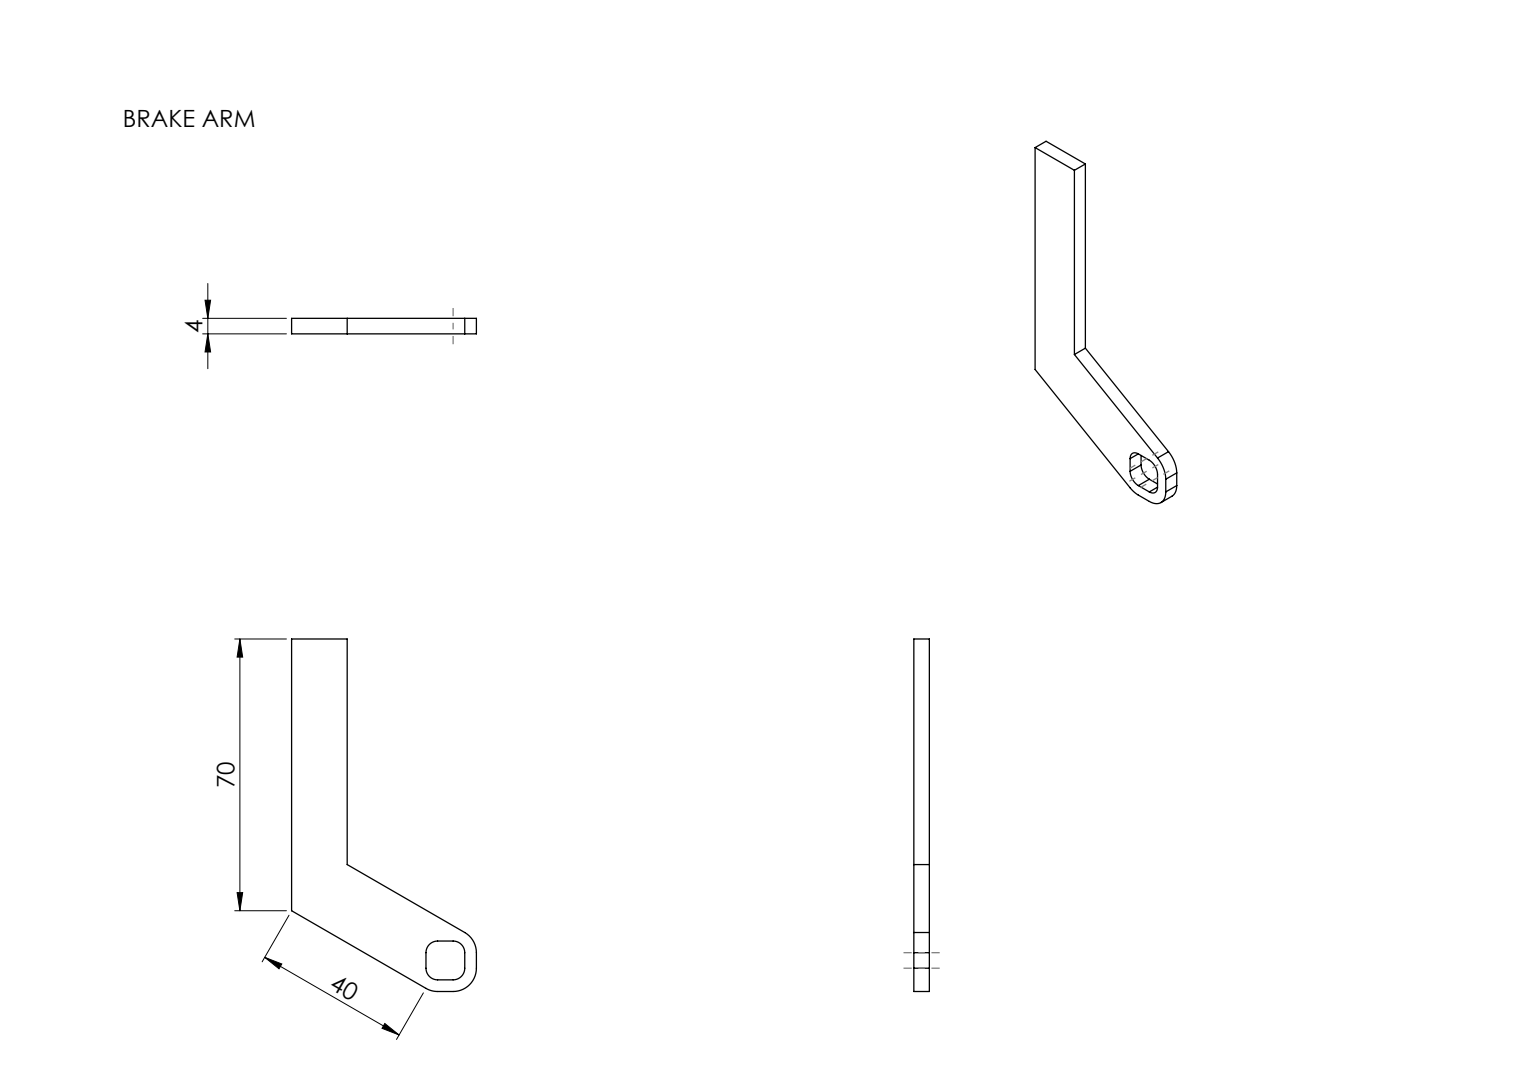
ISO-10303-21;
HEADER;
FILE_DESCRIPTION (('STEP AP214'),
    '1' );
FILE_NAME ('brake arm.step',
    '2026-10-08T05:56:58',
    ( '' ),
    ( '' ),
    'SwSTEP 2.0',
    'SolidWorks 2026',
    '' );
FILE_SCHEMA (( 'AUTOMOTIVE_DESIGN' ));
ENDSEC;

DATA;
#81=AXIS2_PLACEMENT_3D ( 'NONE', #18484, #1485, #6266 ) ;
#85=ORIENTED_EDGE ( 'NONE', *, *, #1576, .T. ) ;
#161=EDGE_LOOP ( 'NONE', ( #14576, #14310, #4192, #11228 ) ) ;
#198=CARTESIAN_POINT ( 'NONE',  ( -2.000000000000000000, 1.999999999999998224, 41.99999999999999289 ) ) ;
#237=EDGE_CURVE ( 'NONE', #6503, #6248, #1744, .T. ) ;
#247=VECTOR ( 'NONE', #10712, 1000.000000000000000 ) ;
#276=EDGE_CURVE ( 'NONE', #11279, #870, #9053, .T. ) ;
#316=CARTESIAN_POINT ( 'NONE',  ( -25.31088913245550032, 24.69615242270646149, 37.99999999999999289 ) ) ;
#333=EDGE_CURVE ( 'NONE', #18696, #7394, #11045, .T. ) ;
#336=COLOUR_RGB ( '', 0.08235294, 0.09019608, 0.10196078) ;
#393=VECTOR ( 'NONE', #16004, 1000.000000000000000 ) ;
#399=EDGE_CURVE ( 'NONE', #17067, #16866, #445, .T. ) ;
#445=LINE ( 'NONE', #1934, #5840 ) ;
#469=AXIS2_PLACEMENT_3D ( 'NONE', #3938, #11542, #11357 ) ;
#506=ORIENTED_EDGE ( 'NONE', *, *, #18779, .F. ) ;
#580=CARTESIAN_POINT ( 'NONE',  ( 5.000000000000000000, 1.999999999999998224, 37.99999999999999289 ) ) ;
#596=CIRCLE ( 'NONE', #10178, 3.000000000000000000 ) ;
#602=CARTESIAN_POINT ( 'NONE',  ( -39.64101615137757761, -1.650388831904890594E-13, 37.99999999999999289 ) ) ;
#648=CARTESIAN_POINT ( 'NONE',  ( -39.64101615137763446, 12.80384757729311573, 37.99999999999999289 ) ) ;
#651=FACE_OUTER_BOUND ( 'NONE', #5044, .T. ) ;
#673=AXIS2_PLACEMENT_3D ( 'NONE', #19698, #12103, #2886 ) ;
#687=ORIENTED_EDGE ( 'NONE', *, *, #13822, .F. ) ;
#690=CARTESIAN_POINT ( 'NONE',  ( 2.000000000000000000, -2.000000000000002665, 37.99999999999999289 ) ) ;
#692=LINE ( 'NONE', #10095, #9730 ) ;
#698=ORIENTED_EDGE ( 'NONE', *, *, #15318, .F. ) ;
#706=LINE ( 'NONE', #3697, #393 ) ;
#809=VERTEX_POINT ( 'NONE', #13215 ) ;
#817=VECTOR ( 'NONE', #17686, 1000.000000000000000 ) ;
#822=PRESENTATION_STYLE_ASSIGNMENT (( #14625 ) ) ;
#824=EDGE_LOOP ( 'NONE', ( #14773, #17764, #4685, #8934 ) ) ;
#828=ORIENTED_EDGE ( 'NONE', *, *, #12966, .F. ) ;
#839=ORIENTED_EDGE ( 'NONE', *, *, #19666, .F. ) ;
#856=CARTESIAN_POINT ( 'NONE',  ( 2.000000000000000000, 1.999999999999998224, 37.99999999999999289 ) ) ;
#870=VERTEX_POINT ( 'NONE', #16016 ) ;
#940=PLANE ( 'NONE',  #17390 ) ;
#1010=EDGE_CURVE ( 'NONE', #11279, #809, #19496, .T. ) ;
#1031=FACE_OUTER_BOUND ( 'NONE', #12382, .T. ) ;
#1082=PRODUCT_DEFINITION_SHAPE ( 'NONE', 'NONE',  #11510 ) ;
#1174=AXIS2_PLACEMENT_3D ( 'NONE', #14507, #5380, #8288 ) ;
#1205=EDGE_CURVE ( 'NONE', #10763, #9786, #692, .T. ) ;
#1214=EDGE_CURVE ( 'NONE', #11454, #10545, #2469, .T. ) ;
#1229=CARTESIAN_POINT ( 'NONE',  ( -3.207603742328077057E-13, 82.80384757729329692, 37.99999999999999289 ) ) ;
#1269=CARTESIAN_POINT ( 'NONE',  ( 1.999999999999998668, -8.000000000000003553, 37.99999999999999289 ) ) ;
#1345=CARTESIAN_POINT ( 'NONE',  ( -0.000000000000000000, -8.000000000000003553, 37.99999999999999289 ) ) ;
#1353=LINE ( 'NONE', #7228, #12881 ) ;
#1391=EDGE_CURVE ( 'NONE', #11279, #5905, #4283, .T. ) ;
#1400=EDGE_CURVE ( 'NONE', #8532, #2993, #16980, .T. ) ;
#1403=DIRECTION ( 'NONE',  ( 0.000000000000000000, 0.000000000000000000, 1.000000000000000000 ) ) ;
#1419=CARTESIAN_POINT ( 'NONE',  ( 2.000000000000000000, 4.999999999999998224, 37.99999999999999289 ) ) ;
#1420=CARTESIAN_POINT ( 'NONE',  ( -2.000000000000000000, -2.000000000000002665, 41.99999999999999289 ) ) ;
#1425=ORIENTED_EDGE ( 'NONE', *, *, #18491, .F. ) ;
#1448=VERTEX_POINT ( 'NONE', #17551 ) ;
#1485=DIRECTION ( 'NONE',  ( -0.000000000000000000, 0.000000000000000000, 1.000000000000000000 ) ) ;
#1518=DIRECTION ( 'NONE',  ( 1.000000000000000000, 0.000000000000000000, 0.000000000000000000 ) ) ;
#1530=LINE ( 'NONE', #10535, #6369 ) ;
#1576=EDGE_CURVE ( 'NONE', #10781, #5905, #18332, .T. ) ;
#1589=ADVANCED_FACE ( 'NONE', ( #9131 ), #7404, .F. ) ;
#1636=LINE ( 'NONE', #9245, #19000 ) ;
#1649=VECTOR ( 'NONE', #1909, 1000.000000000000000 ) ;
#1656=EDGE_LOOP ( 'NONE', ( #14226, #10077, #1425, #11923 ) ) ;
#1719=ADVANCED_FACE ( 'NONE', ( #2114, #8217 ), #17429, .F. ) ;
#1721=LINE ( 'NONE', #13417, #11250 ) ;
#1744=LINE ( 'NONE', #1345, #15759 ) ;
#1806=CARTESIAN_POINT ( 'NONE',  ( -39.64101615137757761, -1.650388831904890594E-13, 41.99999999999999289 ) ) ;
#1839=DIRECTION ( 'NONE',  ( 0.000000000000000000, 0.000000000000000000, 1.000000000000000000 ) ) ;
#1864=DIRECTION ( 'NONE',  ( 0.000000000000000000, 0.000000000000000000, 1.000000000000000000 ) ) ;
#1865=DIRECTION ( 'NONE',  ( -0.000000000000000000, 0.000000000000000000, 1.000000000000000000 ) ) ;
#1871=ORIENTED_EDGE ( 'NONE', *, *, #12830, .T. ) ;
#1905=CARTESIAN_POINT ( 'NONE',  ( -5.000000000000000000, 1.999999999999998668, 41.99999999999999289 ) ) ;
#1909=DIRECTION ( 'NONE',  ( 1.000000000000000000, 0.000000000000000000, 0.000000000000000000 ) ) ;
#1934=CARTESIAN_POINT ( 'NONE',  ( 5.000000000000000000, 0.000000000000000000, 37.99999999999999289 ) ) ;
#1945=ORIENTED_EDGE ( 'NONE', *, *, #9793, .T. ) ;
#1948=DIRECTION ( 'NONE',  ( -0.4999999999999947820, -0.8660254037844417052, 0.000000000000000000 ) ) ;
#2051=EDGE_CURVE ( 'NONE', #5844, #14373, #5895, .T. ) ;
#2054=AXIS2_PLACEMENT_3D ( 'NONE', #11449, #14251, #3640 ) ;
#2057=CARTESIAN_POINT ( 'NONE',  ( 8.000000000000000000, 0.000000000000000000, 37.99999999999999289 ) ) ;
#2111=DIRECTION ( 'NONE',  ( -0.000000000000000000, 0.000000000000000000, 1.000000000000000000 ) ) ;
#2114=FACE_OUTER_BOUND ( 'NONE', #7651, .T. ) ;
#2151=DIRECTION ( 'NONE',  ( 0.000000000000000000, 0.000000000000000000, 1.000000000000000000 ) ) ;
#2271=EDGE_CURVE ( 'NONE', #12858, #1448, #6969, .T. ) ;
#2332=( GEOMETRIC_REPRESENTATION_CONTEXT ( 3 ) GLOBAL_UNCERTAINTY_ASSIGNED_CONTEXT ( ( #11792 ) ) GLOBAL_UNIT_ASSIGNED_CONTEXT ( ( #9933, #11707, #16020 ) ) REPRESENTATION_CONTEXT ( 'NONE', 'WORKASPACE' ) );
#2334=CARTESIAN_POINT ( 'NONE',  ( 1.999999999999999556, -5.000000000000001776, 41.99999999999999289 ) ) ;
#2367=AXIS2_PLACEMENT_3D ( 'NONE', #12036, #18138, #4424 ) ;
#2398=VECTOR ( 'NONE', #8181, 1000.000000000000000 ) ;
#2410=DIRECTION ( 'NONE',  ( 1.000000000000000000, 0.000000000000000000, 0.000000000000000000 ) ) ;
#2434=ORIENTED_EDGE ( 'NONE', *, *, #17702, .T. ) ;
#2435=DIRECTION ( 'NONE',  ( 0.000000000000000000, 0.000000000000000000, 1.000000000000000000 ) ) ;
#2441=EDGE_CURVE ( 'NONE', #8277, #15013, #7462, .T. ) ;
#2469=LINE ( 'NONE', #8677, #7463 ) ;
#2498=CARTESIAN_POINT ( 'NONE',  ( -3.207603742328077057E-13, 82.80384757729329692, 41.99999999999999289 ) ) ;
#2515=ADVANCED_FACE ( 'NONE', ( #14276 ), #15385, .T. ) ;
#2527=ORIENTED_EDGE ( 'NONE', *, *, #1214, .F. ) ;
#2552=AXIS2_PLACEMENT_3D ( 'NONE', #15435, #15728, #18430 ) ;
#2653=DIRECTION ( 'NONE',  ( -1.000000000000000000, 0.000000000000000000, -0.000000000000000000 ) ) ;
#2661=CARTESIAN_POINT ( 'NONE',  ( -39.64101615137792578, 82.80384757729314060, 37.99999999999999289 ) ) ;
#2737=CIRCLE ( 'NONE', #5306, 3.000000000000000000 ) ;
#2753=ORIENTED_EDGE ( 'NONE', *, *, #8979, .F. ) ;
#2755=FACE_OUTER_BOUND ( 'NONE', #18781, .T. ) ;
#2758=CARTESIAN_POINT ( 'NONE',  ( 1.999999999999999556, -5.000000000000001776, 37.99999999999999289 ) ) ;
#2886=DIRECTION ( 'NONE',  ( 1.000000000000000000, 0.000000000000000000, 0.000000000000000000 ) ) ;
#2904=VERTEX_POINT ( 'NONE', #7020 ) ;
#2912=ORIENTED_EDGE ( 'NONE', *, *, #2271, .F. ) ;
#2942=ORIENTED_EDGE ( 'NONE', *, *, #1205, .F. ) ;
#2943=PLANE ( 'NONE',  #14850 ) ;
#2955=EDGE_LOOP ( 'NONE', ( #4427, #15410, #16999, #3356 ) ) ;
#2970=AXIS2_PLACEMENT_3D ( 'NONE', #8264, #6744, #13554 ) ;
#2989=CYLINDRICAL_SURFACE ( 'NONE', #673, 3.000000000000000000 ) ;
#2993=VERTEX_POINT ( 'NONE', #7594 ) ;
#3010=ORIENTED_EDGE ( 'NONE', *, *, #19158, .T. ) ;
#3036=DIRECTION ( 'NONE',  ( 0.000000000000000000, 0.000000000000000000, 1.000000000000000000 ) ) ;
#3046=ORIENTED_EDGE ( 'NONE', *, *, #13258, .T. ) ;
#3074=CARTESIAN_POINT ( 'NONE',  ( -2.000000000000000000, -2.000000000000001776, 37.99999999999999289 ) ) ;
#3107=CARTESIAN_POINT ( 'NONE',  ( -4.366025403784388637, -7.562177826491097044, 41.99999999999999289 ) ) ;
#3120=ADVANCED_FACE ( 'NONE', ( #18799 ), #3498, .F. ) ;
#3202=AXIS2_PLACEMENT_3D ( 'NONE', #4187, #14895, #8689 ) ;
#3233=VECTOR ( 'NONE', #10284, 1000.000000000000000 ) ;
#3270=DIRECTION ( 'NONE',  ( 1.000000000000000000, 0.000000000000000000, 0.000000000000000000 ) ) ;
#3356=ORIENTED_EDGE ( 'NONE', *, *, #18779, .T. ) ;
#3467=ORIENTED_EDGE ( 'NONE', *, *, #9342, .T. ) ;
#3498=PLANE ( 'NONE',  #10025 ) ;
#3508=VECTOR ( 'NONE', #9064, 1000.000000000000000 ) ;
#3602=VERTEX_POINT ( 'NONE', #14726 ) ;
#3615=CARTESIAN_POINT ( 'NONE',  ( 0.000000000000000000, 0.000000000000000000, 37.99999999999999289 ) ) ;
#3640=DIRECTION ( 'NONE',  ( 1.000000000000000000, 0.000000000000000000, 0.000000000000000000 ) ) ;
#3641=VECTOR ( 'NONE', #10871, 1000.000000000000000 ) ;
#3658=LINE ( 'NONE', #18764, #5710 ) ;
#3659=PLANE ( 'NONE',  #2970 ) ;
#3697=CARTESIAN_POINT ( 'NONE',  ( -25.31088913245550032, 24.69615242270646149, 37.99999999999999289 ) ) ;
#3714=DIRECTION ( 'NONE',  ( -0.000000000000000000, 0.000000000000000000, 1.000000000000000000 ) ) ;
#3716=DIRECTION ( 'NONE',  ( 1.000000000000000000, 3.873737557103174326E-15, 0.000000000000000000 ) ) ;
#3722=EDGE_CURVE ( 'NONE', #17625, #10948, #5699, .T. ) ;
#3755=AXIS2_PLACEMENT_3D ( 'NONE', #856, #5633, #5727 ) ;
#3807=CARTESIAN_POINT ( 'NONE',  ( -4.999999999999966249, -7.196152422706654228, 37.99999999999999289 ) ) ;
#3837=CIRCLE ( 'NONE', #2552, 6.000000000000000000 ) ;
#3872=ORIENTED_EDGE ( 'NONE', *, *, #16483, .T. ) ;
#3883=SURFACE_STYLE_USAGE ( .BOTH. , #11303 ) ;
#3897=PLANE ( 'NONE',  #7220 ) ;
#3938=CARTESIAN_POINT ( 'NONE',  ( 0.000000000000000000, 4.999999999999998224, 37.99999999999999289 ) ) ;
#3959=EDGE_CURVE ( 'NONE', #15013, #1448, #7142, .T. ) ;
#3999=LINE ( 'NONE', #16303, #15549 ) ;
#4009=CYLINDRICAL_SURFACE ( 'NONE', #5615, 3.000000000000000000 ) ;
#4034=CARTESIAN_POINT ( 'NONE',  ( -5.000000000000000000, -2.000000000000001332, 37.99999999999999289 ) ) ;
#4146=ADVANCED_FACE ( 'NONE', ( #9470 ), #15767, .F. ) ;
#4150=EDGE_CURVE ( 'NONE', #11541, #11454, #9876, .T. ) ;
#4167=ORIENTED_EDGE ( 'NONE', *, *, #237, .T. ) ;
#4182=ORIENTED_EDGE ( 'NONE', *, *, #333, .F. ) ;
#4187=CARTESIAN_POINT ( 'NONE',  ( 2.000000000000000000, -2.000000000000001776, 37.99999999999999289 ) ) ;
#4192=ORIENTED_EDGE ( 'NONE', *, *, #9827, .F. ) ;
#4215=DIRECTION ( 'NONE',  ( 0.000000000000000000, 0.000000000000000000, 1.000000000000000000 ) ) ;
#4266=ADVANCED_FACE ( 'NONE', ( #19441 ), #14566, .F. ) ;
#4283=CIRCLE ( 'NONE', #2054, 6.000000000000000000 ) ;
#4320=ADVANCED_FACE ( 'NONE', ( #8553 ), #11648, .T. ) ;
#4364=VECTOR ( 'NONE', #15110, 1000.000000000000000 ) ;
#4402=DIRECTION ( 'NONE',  ( 0.000000000000000000, -1.000000000000000000, 0.000000000000000000 ) ) ;
#4424=DIRECTION ( 'NONE',  ( 4.060088635510494296E-15, -1.000000000000000000, 0.000000000000000000 ) ) ;
#4427=ORIENTED_EDGE ( 'NONE', *, *, #10847, .T. ) ;
#4510=CIRCLE ( 'NONE', #16022, 6.000000000000000000 ) ;
#4528=EDGE_CURVE ( 'NONE', #809, #2904, #13228, .T. ) ;
#4578=DIRECTION ( 'NONE',  ( 0.000000000000000000, 0.000000000000000000, 1.000000000000000000 ) ) ;
#4606=LINE ( 'NONE', #16518, #247 ) ;
#4613=EDGE_CURVE ( 'NONE', #7394, #2993, #15324, .T. ) ;
#4681=CARTESIAN_POINT ( 'NONE',  ( 5.000000000000000000, -2.000000000000001776, 37.99999999999999289 ) ) ;
#4685=ORIENTED_EDGE ( 'NONE', *, *, #19313, .F. ) ;
#4793=EDGE_CURVE ( 'NONE', #2993, #6802, #18806, .T. ) ;
#4813=ORIENTED_EDGE ( 'NONE', *, *, #11062, .F. ) ;
#4853=ORIENTED_EDGE ( 'NONE', *, *, #18375, .F. ) ;
#4865=VECTOR ( 'NONE', #9909, 1000.000000000000000 ) ;
#4897=DIRECTION ( 'NONE',  ( -0.000000000000000000, 0.000000000000000000, 1.000000000000000000 ) ) ;
#4959=VERTEX_POINT ( 'NONE', #19780 ) ;
#5044=EDGE_LOOP ( 'NONE', ( #10868, #6394, #19620, #6401 ) ) ;
#5076=CARTESIAN_POINT ( 'NONE',  ( 4.999999999999963585, 7.196152422706642682, 41.99999999999999289 ) ) ;
#5088=DIRECTION ( 'NONE',  ( 1.000000000000000000, 4.163336342344335449E-15, -0.000000000000000000 ) ) ;
#5094=CARTESIAN_POINT ( 'NONE',  ( -4.999999999999966249, -7.196152422706654228, 41.99999999999999289 ) ) ;
#5098=AXIS2_PLACEMENT_3D ( 'NONE', #10127, #8524, #2410 ) ;
#5214=DIRECTION ( 'NONE',  ( 1.000000000000000000, 0.000000000000000000, 0.000000000000000000 ) ) ;
#5269=ADVANCED_FACE ( 'NONE', ( #2755 ), #19762, .F. ) ;
#5306=AXIS2_PLACEMENT_3D ( 'NONE', #13621, #10429, #13919 ) ;
#5355=VECTOR ( 'NONE', #19715, 1000.000000000000000 ) ;
#5380=DIRECTION ( 'NONE',  ( 3.873737557103174326E-15, -1.000000000000000000, 0.000000000000000000 ) ) ;
#5446=MECHANICAL_DESIGN_GEOMETRIC_PRESENTATION_REPRESENTATION('',(#15990),#7964);
#5465=AXIS2_PLACEMENT_3D ( 'NONE', #690, #6768, #15896 ) ;
#5487=VECTOR ( 'NONE', #4578, 1000.000000000000000 ) ;
#5513=ORIENTED_EDGE ( 'NONE', *, *, #9678, .T. ) ;
#5518=VECTOR ( 'NONE', #1839, 1000.000000000000000 ) ;
#5579=CYLINDRICAL_SURFACE ( 'NONE', #3202, 3.000000000000000000 ) ;
#5594=( NAMED_UNIT ( * ) SI_UNIT ( $, .STERADIAN. ) SOLID_ANGLE_UNIT ( ) );
#5600=ORIENTED_EDGE ( 'NONE', *, *, #9678, .F. ) ;
#5615=AXIS2_PLACEMENT_3D ( 'NONE', #11422, #8215, #6798 ) ;
#5633=DIRECTION ( 'NONE',  ( 0.000000000000000000, 0.000000000000000000, 1.000000000000000000 ) ) ;
#5657=EDGE_CURVE ( 'NONE', #7394, #3602, #17136, .T. ) ;
#5666=EDGE_CURVE ( 'NONE', #10545, #17625, #2737, .T. ) ;
#5674=CIRCLE ( 'NONE', #8246, 3.000000000000000000 ) ;
#5697=ORIENTED_EDGE ( 'NONE', *, *, #10847, .F. ) ;
#5699=LINE ( 'NONE', #13313, #13011 ) ;
#5710=VECTOR ( 'NONE', #1864, 1000.000000000000000 ) ;
#5727=DIRECTION ( 'NONE',  ( 1.000000000000000000, 0.000000000000000000, 0.000000000000000000 ) ) ;
#5741=DIRECTION ( 'NONE',  ( 0.000000000000000000, 0.000000000000000000, 1.000000000000000000 ) ) ;
#5809=DIRECTION ( 'NONE',  ( -1.000000000000000000, 0.000000000000000000, 0.000000000000000000 ) ) ;
#5818=ORIENTED_EDGE ( 'NONE', *, *, #7312, .T. ) ;
#5840=VECTOR ( 'NONE', #10947, 1000.000000000000000 ) ;
#5844=VERTEX_POINT ( 'NONE', #1905 ) ;
#5895=LINE ( 'NONE', #18113, #10388 ) ;
#5905=VERTEX_POINT ( 'NONE', #14215 ) ;
#5992=EDGE_CURVE ( 'NONE', #8277, #12858, #3999, .T. ) ;
#6012=CARTESIAN_POINT ( 'NONE',  ( 4.366025403784385972, 7.562177826491085497, 37.99999999999999289 ) ) ;
#6021=DIRECTION ( 'NONE',  ( 1.000000000000000000, 0.000000000000000000, 0.000000000000000000 ) ) ;
#6057=ADVANCED_FACE ( 'NONE', ( #17609 ), #3897, .F. ) ;
#6063=EDGE_CURVE ( 'NONE', #12858, #18724, #14597, .T. ) ;
#6115=DIRECTION ( 'NONE',  ( 1.000000000000000000, 3.873737557103174326E-15, 0.000000000000000000 ) ) ;
#6152=VECTOR ( 'NONE', #14884, 1000.000000000000000 ) ;
#6206=EDGE_LOOP ( 'NONE', ( #3046, #11436, #5600, #6318 ) ) ;
#6207=CARTESIAN_POINT ( 'NONE',  ( -25.31088913245550032, 24.69615242270646149, 41.99999999999999289 ) ) ;
#6230=DIRECTION ( 'NONE',  ( 1.000000000000000000, 0.000000000000000000, 0.000000000000000000 ) ) ;
#6248=VERTEX_POINT ( 'NONE', #11289 ) ;
#6266=DIRECTION ( 'NONE',  ( 1.000000000000000000, 0.000000000000000000, 0.000000000000000000 ) ) ;
#6318=ORIENTED_EDGE ( 'NONE', *, *, #12966, .T. ) ;
#6344=EDGE_LOOP ( 'NONE', ( #19742, #9446, #9633, #18836 ) ) ;
#6369=VECTOR ( 'NONE', #10441, 1000.000000000000000 ) ;
#6394=ORIENTED_EDGE ( 'NONE', *, *, #15285, .F. ) ;
#6401=ORIENTED_EDGE ( 'NONE', *, *, #10994, .T. ) ;
#6483=EDGE_CURVE ( 'NONE', #12253, #10545, #11975, .T. ) ;
#6503=VERTEX_POINT ( 'NONE', #1269 ) ;
#6528=ORIENTED_EDGE ( 'NONE', *, *, #15670, .F. ) ;
#6548=CARTESIAN_POINT ( 'NONE',  ( 2.000000000000000000, -2.000000000000002665, 37.99999999999999289 ) ) ;
#6562=LINE ( 'NONE', #8385, #2398 ) ;
#6564=AXIS2_PLACEMENT_3D ( 'NONE', #17715, #2111, #19207 ) ;
#6571=PLANE ( 'NONE',  #1174 ) ;
#6574=ORIENTED_EDGE ( 'NONE', *, *, #3722, .T. ) ;
#6654=VECTOR ( 'NONE', #2435, 1000.000000000000000 ) ;
#6671=FACE_OUTER_BOUND ( 'NONE', #18548, .T. ) ;
#6674=FILL_AREA_STYLE_COLOUR ( '', #336 ) ;
#6734=DIRECTION ( 'NONE',  ( 0.8660254037844417052, -0.4999999999999947820, 0.000000000000000000 ) ) ;
#6737=EDGE_CURVE ( 'NONE', #4959, #2904, #4510, .T. ) ;
#6744=DIRECTION ( 'NONE',  ( 0.4999999999999945044, 0.8660254037844419273, -0.000000000000000000 ) ) ;
#6768=DIRECTION ( 'NONE',  ( -0.000000000000000000, 0.000000000000000000, 1.000000000000000000 ) ) ;
#6770=DIRECTION ( 'NONE',  ( 0.8660254037844417052, -0.4999999999999947820, 0.000000000000000000 ) ) ;
#6772=CIRCLE ( 'NONE', #14145, 3.000000000000000000 ) ;
#6798=DIRECTION ( 'NONE',  ( 1.000000000000000000, 0.000000000000000000, 0.000000000000000000 ) ) ;
#6802=VERTEX_POINT ( 'NONE', #9038 ) ;
#6969=LINE ( 'NONE', #19183, #4865 ) ;
#6973=UNCERTAINTY_MEASURE_WITH_UNIT (LENGTH_MEASURE( 1.000000000000000082E-05 ), #15700, 'distance_accuracy_value', 'NONE');
#6994=DIRECTION ( 'NONE',  ( 0.000000000000000000, 0.000000000000000000, 1.000000000000000000 ) ) ;
#7020=CARTESIAN_POINT ( 'NONE',  ( 8.000000000000000000, -2.000000000000002665, 41.99999999999999289 ) ) ;
#7026=CARTESIAN_POINT ( 'NONE',  ( 2.000000000000000000, 1.999999999999997335, 37.99999999999999289 ) ) ;
#7091=FACE_BOUND ( 'NONE', #9946, .T. ) ;
#7142=LINE ( 'NONE', #16476, #11425 ) ;
#7182=( NAMED_UNIT ( * ) PLANE_ANGLE_UNIT ( ) SI_UNIT ( $, .RADIAN. ) );
#7220=AXIS2_PLACEMENT_3D ( 'NONE', #16212, #11798, #8599 ) ;
#7228=CARTESIAN_POINT ( 'NONE',  ( -5.000000000000000000, 0.000000000000000000, 37.99999999999999289 ) ) ;
#7247=EDGE_LOOP ( 'NONE', ( #19691, #506, #839, #3872 ) ) ;
#7277=CARTESIAN_POINT ( 'NONE',  ( 8.000000000000000000, 0.000000000000000000, 37.99999999999999289 ) ) ;
#7312=EDGE_CURVE ( 'NONE', #10781, #10763, #706, .T. ) ;
#7320=CARTESIAN_POINT ( 'NONE',  ( -25.31088913245573835, 82.80384757729319745, 37.99999999999999289 ) ) ;
#7370=APPLICATION_CONTEXT ( 'automotive_design' ) ;
#7394=VERTEX_POINT ( 'NONE', #5094 ) ;
#7404=PLANE ( 'NONE',  #2367 ) ;
#7414=LINE ( 'NONE', #16166, #6654 ) ;
#7462=LINE ( 'NONE', #10393, #5487 ) ;
#7463=VECTOR ( 'NONE', #12796, 1000.000000000000000 ) ;
#7499=ORIENTED_EDGE ( 'NONE', *, *, #6737, .T. ) ;
#7502=AXIS2_PLACEMENT_3D ( 'NONE', #14084, #9202, #18490 ) ;
#7528=EDGE_CURVE ( 'NONE', #18696, #6248, #16697, .T. ) ;
#7532=EDGE_LOOP ( 'NONE', ( #17572, #13360, #2753, #9335 ) ) ;
#7544=CARTESIAN_POINT ( 'NONE',  ( 2.000000000000000000, 1.999999999999998224, 41.99999999999999289 ) ) ;
#7594=CARTESIAN_POINT ( 'NONE',  ( -39.64101615137763446, 12.80384757729311573, 41.99999999999999289 ) ) ;
#7651=EDGE_LOOP ( 'NONE', ( #3467, #13166, #9459, #15462, #85, #12955, #14346, #14023, #4167, #8073 ) ) ;
#7732=AXIS2_PLACEMENT_3D ( 'NONE', #6548, #18574, #8167 ) ;
#7824=CARTESIAN_POINT ( 'NONE',  ( -5.000000000000000000, 1.999999999999998668, 37.99999999999999289 ) ) ;
#7838=AXIS2_PLACEMENT_3D ( 'NONE', #13670, #16781, #8872 ) ;
#7845=ORIENTED_EDGE ( 'NONE', *, *, #15670, .T. ) ;
#7866=DIRECTION ( 'NONE',  ( -0.000000000000000000, 0.000000000000000000, 1.000000000000000000 ) ) ;
#7874=CIRCLE ( 'NONE', #19066, 3.000000000000000000 ) ;
#7964=( GEOMETRIC_REPRESENTATION_CONTEXT ( 3 ) GLOBAL_UNCERTAINTY_ASSIGNED_CONTEXT ( ( #6973 ) ) GLOBAL_UNIT_ASSIGNED_CONTEXT ( ( #15700, #10004, #16105 ) ) REPRESENTATION_CONTEXT ( 'NONE', 'WORKASPACE' ) );
#8010=ORIENTED_EDGE ( 'NONE', *, *, #1576, .F. ) ;
#8073=ORIENTED_EDGE ( 'NONE', *, *, #7528, .F. ) ;
#8148=SHAPE_DEFINITION_REPRESENTATION ( #1082, #15643 ) ;
#8153=ORIENTED_EDGE ( 'NONE', *, *, #5992, .F. ) ;
#8167=DIRECTION ( 'NONE',  ( 1.000000000000000000, 0.000000000000000000, 0.000000000000000000 ) ) ;
#8181=DIRECTION ( 'NONE',  ( -4.163336342344335449E-15, 1.000000000000000000, 0.000000000000000000 ) ) ;
#8215=DIRECTION ( 'NONE',  ( 0.000000000000000000, 0.000000000000000000, 1.000000000000000000 ) ) ;
#8217=FACE_BOUND ( 'NONE', #19173, .T. ) ;
#8246=AXIS2_PLACEMENT_3D ( 'NONE', #3074, #7866, #3270 ) ;
#8264=CARTESIAN_POINT ( 'NONE',  ( -4.366025403784388637, -7.562177826491097044, 37.99999999999999289 ) ) ;
#8277=VERTEX_POINT ( 'NONE', #1419 ) ;
#8288=DIRECTION ( 'NONE',  ( 1.000000000000000000, 3.873737557103174326E-15, 0.000000000000000000 ) ) ;
#8306=ORIENTED_EDGE ( 'NONE', *, *, #399, .T. ) ;
#8317=LINE ( 'NONE', #2498, #15021 ) ;
#8345=CARTESIAN_POINT ( 'NONE',  ( 0.000000000000000000, -8.000000000000003553, 37.99999999999999289 ) ) ;
#8355=CARTESIAN_POINT ( 'NONE',  ( 4.366025403784385972, 7.562177826491085497, 37.99999999999999289 ) ) ;
#8385=CARTESIAN_POINT ( 'NONE',  ( -39.64101615137757761, -1.650388831904890594E-13, 37.99999999999999289 ) ) ;
#8453=PLANE ( 'NONE',  #469 ) ;
#8489=CARTESIAN_POINT ( 'NONE',  ( 4.999999999999963585, 7.196152422706642682, 37.99999999999999289 ) ) ;
#8511=ORIENTED_EDGE ( 'NONE', *, *, #6063, .F. ) ;
#8524=DIRECTION ( 'NONE',  ( -0.000000000000000000, 0.000000000000000000, 1.000000000000000000 ) ) ;
#8532=VERTEX_POINT ( 'NONE', #16302 ) ;
#8549=ORIENTED_EDGE ( 'NONE', *, *, #19313, .T. ) ;
#8553=FACE_OUTER_BOUND ( 'NONE', #12626, .T. ) ;
#8599=DIRECTION ( 'NONE',  ( 0.000000000000000000, -0.000000000000000000, -1.000000000000000000 ) ) ;
#8600=AXIS2_PLACEMENT_3D ( 'NONE', #2057, #15872, #11171 ) ;
#8654=DIRECTION ( 'NONE',  ( 0.000000000000000000, -1.000000000000000000, 0.000000000000000000 ) ) ;
#8677=CARTESIAN_POINT ( 'NONE',  ( 0.000000000000000000, -5.000000000000001776, 41.99999999999999289 ) ) ;
#8689=DIRECTION ( 'NONE',  ( 1.000000000000000000, 0.000000000000000000, 0.000000000000000000 ) ) ;
#8729=STYLED_ITEM ( 'NONE', ( #822 ), #10191 ) ;
#8751=CLOSED_SHELL ( 'NONE', ( #14882, #17525, #6057, #16932, #5269, #4266, #15195, #19573, #3120, #11263, #1589, #4146, #4320, #13846, #2515, #15239, #15629, #10796, #1719, #16635 ) ) ;
#8798=DIRECTION ( 'NONE',  ( 1.000000000000000000, 0.000000000000000000, 0.000000000000000000 ) ) ;
#8861=DIRECTION ( 'NONE',  ( -1.000000000000000000, 0.000000000000000000, 0.000000000000000000 ) ) ;
#8872=DIRECTION ( 'NONE',  ( 0.000000000000000000, 0.000000000000000000, -1.000000000000000000 ) ) ;
#8934=ORIENTED_EDGE ( 'NONE', *, *, #6483, .T. ) ;
#8979=EDGE_CURVE ( 'NONE', #9207, #10781, #17984, .T. ) ;
#9038=CARTESIAN_POINT ( 'NONE',  ( -39.64101615137792578, 82.80384757729314060, 41.99999999999999289 ) ) ;
#9053=LINE ( 'NONE', #15153, #17667 ) ;
#9064=DIRECTION ( 'NONE',  ( 4.060088635510494296E-15, -1.000000000000000000, 0.000000000000000000 ) ) ;
#9131=FACE_OUTER_BOUND ( 'NONE', #7532, .T. ) ;
#9141=CARTESIAN_POINT ( 'NONE',  ( 2.000000000000000000, -2.000000000000002665, 41.99999999999999289 ) ) ;
#9183=CARTESIAN_POINT ( 'NONE',  ( -2.000000000000000000, -5.000000000000001776, 37.99999999999999289 ) ) ;
#9202=DIRECTION ( 'NONE',  ( -0.000000000000000000, 0.000000000000000000, 1.000000000000000000 ) ) ;
#9207=VERTEX_POINT ( 'NONE', #7320 ) ;
#9232=DIRECTION ( 'NONE',  ( 0.8660254037844417052, -0.4999999999999947820, 0.000000000000000000 ) ) ;
#9245=CARTESIAN_POINT ( 'NONE',  ( -4.366025403784388637, -7.562177826491097044, 37.99999999999999289 ) ) ;
#9268=ORIENTED_EDGE ( 'NONE', *, *, #10994, .F. ) ;
#9278=ORIENTED_EDGE ( 'NONE', *, *, #3959, .T. ) ;
#9335=ORIENTED_EDGE ( 'NONE', *, *, #13822, .T. ) ;
#9342=EDGE_CURVE ( 'NONE', #18696, #8532, #1636, .T. ) ;
#9446=ORIENTED_EDGE ( 'NONE', *, *, #1400, .F. ) ;
#9451=ORIENTED_EDGE ( 'NONE', *, *, #276, .F. ) ;
#9459=ORIENTED_EDGE ( 'NONE', *, *, #15318, .T. ) ;
#9470=FACE_OUTER_BOUND ( 'NONE', #9849, .T. ) ;
#9473=CIRCLE ( 'NONE', #6564, 3.000000000000000000 ) ;
#9477=PLANE ( 'NONE',  #8600 ) ;
#9527=CARTESIAN_POINT ( 'NONE',  ( 0.000000000000000000, -5.000000000000001776, 37.99999999999999289 ) ) ;
#9633=ORIENTED_EDGE ( 'NONE', *, *, #9342, .F. ) ;
#9661=PRODUCT_CONTEXT ( 'NONE', #17626, 'mechanical' ) ;
#9665=ORIENTED_EDGE ( 'NONE', *, *, #4613, .F. ) ;
#9678=EDGE_CURVE ( 'NONE', #16866, #8277, #18061, .T. ) ;
#9730=VECTOR ( 'NONE', #6770, 1000.000000000000000 ) ;
#9764=DIRECTION ( 'NONE',  ( 0.000000000000000000, 1.000000000000000000, -0.000000000000000000 ) ) ;
#9786=VERTEX_POINT ( 'NONE', #5076 ) ;
#9793=EDGE_CURVE ( 'NONE', #5905, #9786, #16194, .T. ) ;
#9827=EDGE_CURVE ( 'NONE', #8532, #9982, #6562, .T. ) ;
#9833=DIRECTION ( 'NONE',  ( 0.000000000000000000, 0.000000000000000000, 1.000000000000000000 ) ) ;
#9849=EDGE_LOOP ( 'NONE', ( #14208, #10384, #8010, #5818 ) ) ;
#9860=ORIENTED_EDGE ( 'NONE', *, *, #5657, .F. ) ;
#9876=LINE ( 'NONE', #15866, #12394 ) ;
#9909=DIRECTION ( 'NONE',  ( 0.000000000000000000, 0.000000000000000000, 1.000000000000000000 ) ) ;
#9933=( LENGTH_UNIT ( ) NAMED_UNIT ( * ) SI_UNIT ( .MILLI., .METRE. ) );
#9946=EDGE_LOOP ( 'NONE', ( #18551, #4813, #16973, #12179, #13079, #18330, #2527, #5697 ) ) ;
#9982=VERTEX_POINT ( 'NONE', #2661 ) ;
#10004=( NAMED_UNIT ( * ) PLANE_ANGLE_UNIT ( ) SI_UNIT ( $, .RADIAN. ) );
#10025=AXIS2_PLACEMENT_3D ( 'NONE', #602, #5088, #11306 ) ;
#10077=ORIENTED_EDGE ( 'NONE', *, *, #6483, .F. ) ;
#10095=CARTESIAN_POINT ( 'NONE',  ( 4.366025403784385972, 7.562177826491085497, 41.99999999999999289 ) ) ;
#10127=CARTESIAN_POINT ( 'NONE',  ( 0.000000000000000000, 0.000000000000000000, 41.99999999999999289 ) ) ;
#10166=VECTOR ( 'NONE', #4215, 1000.000000000000000 ) ;
#10178=AXIS2_PLACEMENT_3D ( 'NONE', #7544, #18460, #19758 ) ;
#10191=ADVANCED_BREP_SHAPE_REPRESENTATION ( '', ( #16005, #16724 ), #2332 ) ;
#10206=DIRECTION ( 'NONE',  ( -1.000000000000000000, 0.000000000000000000, -0.000000000000000000 ) ) ;
#10218=SHAPE_REPRESENTATION_RELATIONSHIP ( 'NONE' , 'NONE' ,  #15643, #10191 ) ;
#10284=DIRECTION ( 'NONE',  ( 0.000000000000000000, 0.000000000000000000, 1.000000000000000000 ) ) ;
#10319=CARTESIAN_POINT ( 'NONE',  ( 1.999999999999998668, -8.000000000000003553, 37.99999999999999289 ) ) ;
#10384=ORIENTED_EDGE ( 'NONE', *, *, #9793, .F. ) ;
#10388=VECTOR ( 'NONE', #4402, 1000.000000000000000 ) ;
#10393=CARTESIAN_POINT ( 'NONE',  ( 2.000000000000000000, 4.999999999999998224, 37.99999999999999289 ) ) ;
#10429=DIRECTION ( 'NONE',  ( -0.000000000000000000, 0.000000000000000000, 1.000000000000000000 ) ) ;
#10441=DIRECTION ( 'NONE',  ( 0.000000000000000000, 0.000000000000000000, 1.000000000000000000 ) ) ;
#10479=CARTESIAN_POINT ( 'NONE',  ( -25.31088913245540084, -1.027644533213482535E-13, 37.99999999999999289 ) ) ;
#10485=LINE ( 'NONE', #15082, #6152 ) ;
#10514=VERTEX_POINT ( 'NONE', #4034 ) ;
#10535=CARTESIAN_POINT ( 'NONE',  ( -2.000000000000000000, -8.000000000000003553, 37.99999999999999289 ) ) ;
#10545=VERTEX_POINT ( 'NONE', #2334 ) ;
#10590=PRODUCT_DEFINITION_CONTEXT ( 'detailed design', #7370, 'design' ) ;
#10625=VECTOR ( 'NONE', #16580, 1000.000000000000000 ) ;
#10667=VERTEX_POINT ( 'NONE', #10729 ) ;
#10712=DIRECTION ( 'NONE',  ( 0.000000000000000000, 0.000000000000000000, 1.000000000000000000 ) ) ;
#10729=CARTESIAN_POINT ( 'NONE',  ( -25.31088913245573835, 82.80384757729319745, 41.99999999999999289 ) ) ;
#10757=CARTESIAN_POINT ( 'NONE',  ( -5.000000000000000000, 0.000000000000000000, 37.99999999999999289 ) ) ;
#10763=VERTEX_POINT ( 'NONE', #6207 ) ;
#10781=VERTEX_POINT ( 'NONE', #316 ) ;
#10796=ADVANCED_FACE ( 'NONE', ( #12822 ), #4009, .F. ) ;
#10847=EDGE_CURVE ( 'NONE', #14373, #11454, #9473, .T. ) ;
#10868=ORIENTED_EDGE ( 'NONE', *, *, #18375, .T. ) ;
#10870=CARTESIAN_POINT ( 'NONE',  ( 2.000000000000000000, -2.000000000000001776, 37.99999999999999289 ) ) ;
#10871=DIRECTION ( 'NONE',  ( 0.000000000000000000, 0.000000000000000000, 1.000000000000000000 ) ) ;
#10947=DIRECTION ( 'NONE',  ( 0.000000000000000000, 1.000000000000000000, 0.000000000000000000 ) ) ;
#10948=VERTEX_POINT ( 'NONE', #19303 ) ;
#10994=EDGE_CURVE ( 'NONE', #6503, #4959, #14814, .T. ) ;
#10999=DIRECTION ( 'NONE',  ( 1.000000000000000000, 0.000000000000000000, 0.000000000000000000 ) ) ;
#11045=LINE ( 'NONE', #18544, #5518 ) ;
#11062=EDGE_CURVE ( 'NONE', #1448, #5844, #7874, .T. ) ;
#11069=DIRECTION ( 'NONE',  ( 1.000000000000000000, 0.000000000000000000, 0.000000000000000000 ) ) ;
#11124=DIRECTION ( 'NONE',  ( 1.000000000000000000, 0.000000000000000000, 0.000000000000000000 ) ) ;
#11171=DIRECTION ( 'NONE',  ( 0.000000000000000000, 0.000000000000000000, 1.000000000000000000 ) ) ;
#11209=DIRECTION ( 'NONE',  ( -4.163336342344335449E-15, 1.000000000000000000, 0.000000000000000000 ) ) ;
#11228=ORIENTED_EDGE ( 'NONE', *, *, #1400, .T. ) ;
#11250=VECTOR ( 'NONE', #5809, 1000.000000000000000 ) ;
#11263=ADVANCED_FACE ( 'NONE', ( #6671 ), #6571, .F. ) ;
#11279=VERTEX_POINT ( 'NONE', #14296 ) ;
#11289=CARTESIAN_POINT ( 'NONE',  ( -2.000000000000000000, -8.000000000000003553, 37.99999999999999289 ) ) ;
#11295=( GEOMETRIC_REPRESENTATION_CONTEXT ( 3 ) GLOBAL_UNCERTAINTY_ASSIGNED_CONTEXT ( ( #16396 ) ) GLOBAL_UNIT_ASSIGNED_CONTEXT ( ( #14717, #7182, #5594 ) ) REPRESENTATION_CONTEXT ( 'NONE', 'WORKASPACE' ) );
#11303=SURFACE_SIDE_STYLE ('',( #17595 ) ) ;
#11306=DIRECTION ( 'NONE',  ( -4.163336342344335449E-15, 1.000000000000000000, 0.000000000000000000 ) ) ;
#11334=EDGE_LOOP ( 'NONE', ( #3010, #19309, #12459, #13884 ) ) ;
#11357=DIRECTION ( 'NONE',  ( 0.000000000000000000, 0.000000000000000000, 1.000000000000000000 ) ) ;
#11422=CARTESIAN_POINT ( 'NONE',  ( -2.000000000000000000, 1.999999999999998224, 37.99999999999999289 ) ) ;
#11425=VECTOR ( 'NONE', #2653, 1000.000000000000000 ) ;
#11436=ORIENTED_EDGE ( 'NONE', *, *, #2441, .F. ) ;
#11449=CARTESIAN_POINT ( 'NONE',  ( 2.000000000000000000, 1.999999999999997335, 37.99999999999999289 ) ) ;
#11454=VERTEX_POINT ( 'NONE', #11785 ) ;
#11510=PRODUCT_DEFINITION ( 'UNKNOWN', '', #12757, #10590 ) ;
#11541=VERTEX_POINT ( 'NONE', #9183 ) ;
#11542=DIRECTION ( 'NONE',  ( 0.000000000000000000, 1.000000000000000000, -0.000000000000000000 ) ) ;
#11648=CYLINDRICAL_SURFACE ( 'NONE', #19722, 6.000000000000000000 ) ;
#11707=( NAMED_UNIT ( * ) PLANE_ANGLE_UNIT ( ) SI_UNIT ( $, .RADIAN. ) );
#11785=CARTESIAN_POINT ( 'NONE',  ( -2.000000000000000000, -5.000000000000001776, 41.99999999999999289 ) ) ;
#11792=UNCERTAINTY_MEASURE_WITH_UNIT (LENGTH_MEASURE( 1.000000000000000082E-05 ), #9933, 'distance_accuracy_value', 'NONE');
#11793=FACE_OUTER_BOUND ( 'NONE', #824, .T. ) ;
#11798=DIRECTION ( 'NONE',  ( 0.000000000000000000, -1.000000000000000000, 0.000000000000000000 ) ) ;
#11808=FILL_AREA_STYLE ('',( #17911 ) ) ;
#11923=ORIENTED_EDGE ( 'NONE', *, *, #4150, .T. ) ;
#11975=LINE ( 'NONE', #2758, #3233 ) ;
#12036=CARTESIAN_POINT ( 'NONE',  ( -25.31088913245540084, -1.027644533213482535E-13, 37.99999999999999289 ) ) ;
#12103=DIRECTION ( 'NONE',  ( 0.000000000000000000, 0.000000000000000000, 1.000000000000000000 ) ) ;
#12179=ORIENTED_EDGE ( 'NONE', *, *, #13258, .F. ) ;
#12253=VERTEX_POINT ( 'NONE', #13710 ) ;
#12302=EDGE_CURVE ( 'NONE', #17067, #17625, #4606, .T. ) ;
#12382=EDGE_LOOP ( 'NONE', ( #9278, #2912, #8153, #15364 ) ) ;
#12394=VECTOR ( 'NONE', #2151, 1000.000000000000000 ) ;
#12459=ORIENTED_EDGE ( 'NONE', *, *, #1010, .F. ) ;
#12626=EDGE_LOOP ( 'NONE', ( #12942, #9451, #18655, #1945 ) ) ;
#12723=ORIENTED_EDGE ( 'NONE', *, *, #5992, .T. ) ;
#12757=PRODUCT_DEFINITION_FORMATION_WITH_SPECIFIED_SOURCE ( 'ANY', '', #17533, .NOT_KNOWN. ) ;
#12796=DIRECTION ( 'NONE',  ( 1.000000000000000000, 0.000000000000000000, 0.000000000000000000 ) ) ;
#12822=FACE_OUTER_BOUND ( 'NONE', #13885, .T. ) ;
#12830=EDGE_CURVE ( 'NONE', #10514, #11541, #5674, .T. ) ;
#12858=VERTEX_POINT ( 'NONE', #16989 ) ;
#12881=VECTOR ( 'NONE', #8654, 1000.000000000000000 ) ;
#12891=COLOUR_RGB ( '', 0.08235294, 0.09019608, 0.10196078) ;
#12905=CARTESIAN_POINT ( 'NONE',  ( 5.000000000000000000, 1.999999999999998224, 37.99999999999999289 ) ) ;
#12932=FACE_OUTER_BOUND ( 'NONE', #16582, .T. ) ;
#12942=ORIENTED_EDGE ( 'NONE', *, *, #15494, .F. ) ;
#12955=ORIENTED_EDGE ( 'NONE', *, *, #1391, .F. ) ;
#12966=EDGE_CURVE ( 'NONE', #16866, #10948, #19168, .T. ) ;
#13011=VECTOR ( 'NONE', #18317, 1000.000000000000000 ) ;
#13079=ORIENTED_EDGE ( 'NONE', *, *, #3722, .F. ) ;
#13114=SURFACE_SIDE_STYLE ('',( #14529 ) ) ;
#13152=DIRECTION ( 'NONE',  ( 1.000000000000000000, 0.000000000000000000, 0.000000000000000000 ) ) ;
#13166=ORIENTED_EDGE ( 'NONE', *, *, #9827, .T. ) ;
#13215=CARTESIAN_POINT ( 'NONE',  ( 8.000000000000000000, -2.000000000000002665, 37.99999999999999289 ) ) ;
#13228=LINE ( 'NONE', #13315, #10166 ) ;
#13258=EDGE_CURVE ( 'NONE', #10948, #15013, #596, .T. ) ;
#13312=AXIS2_PLACEMENT_3D ( 'NONE', #17900, #16404, #8798 ) ;
#13313=CARTESIAN_POINT ( 'NONE',  ( 5.000000000000000000, 0.000000000000000000, 41.99999999999999289 ) ) ;
#13315=CARTESIAN_POINT ( 'NONE',  ( 8.000000000000000000, -2.000000000000002665, 37.99999999999999289 ) ) ;
#13360=ORIENTED_EDGE ( 'NONE', *, *, #7312, .F. ) ;
#13398=DIRECTION ( 'NONE',  ( 0.000000000000000000, -1.000000000000000000, 0.000000000000000000 ) ) ;
#13417=CARTESIAN_POINT ( 'NONE',  ( -0.000000000000000000, -8.000000000000003553, 41.99999999999999289 ) ) ;
#13479=ORIENTED_EDGE ( 'NONE', *, *, #11062, .T. ) ;
#13514=MECHANICAL_DESIGN_GEOMETRIC_PRESENTATION_REPRESENTATION('',(#8729),#11295);
#13545=EDGE_CURVE ( 'NONE', #9982, #6802, #7414, .T. ) ;
#13554=DIRECTION ( 'NONE',  ( -0.8660254037844418162, 0.4999999999999944489, 0.000000000000000000 ) ) ;
#13618=AXIS2_PLACEMENT_3D ( 'NONE', #1420, #15025, #1518 ) ;
#13621=CARTESIAN_POINT ( 'NONE',  ( 2.000000000000000000, -2.000000000000001776, 41.99999999999999289 ) ) ;
#13670=CARTESIAN_POINT ( 'NONE',  ( 5.000000000000000000, 0.000000000000000000, 37.99999999999999289 ) ) ;
#13675=ORIENTED_EDGE ( 'NONE', *, *, #19158, .F. ) ;
#13710=CARTESIAN_POINT ( 'NONE',  ( 1.999999999999999556, -5.000000000000001776, 37.99999999999999289 ) ) ;
#13752=ORIENTED_EDGE ( 'NONE', *, *, #15494, .T. ) ;
#13822=EDGE_CURVE ( 'NONE', #9207, #10667, #3658, .T. ) ;
#13846=ADVANCED_FACE ( 'NONE', ( #18470 ), #9477, .F. ) ;
#13851=DIRECTION ( 'NONE',  ( -1.000000000000000000, 0.000000000000000000, 0.000000000000000000 ) ) ;
#13875=ORIENTED_EDGE ( 'NONE', *, *, #16483, .F. ) ;
#13884=ORIENTED_EDGE ( 'NONE', *, *, #276, .T. ) ;
#13885=EDGE_LOOP ( 'NONE', ( #13479, #13875, #8511, #14161 ) ) ;
#13919=DIRECTION ( 'NONE',  ( 1.000000000000000000, 0.000000000000000000, 0.000000000000000000 ) ) ;
#14023=ORIENTED_EDGE ( 'NONE', *, *, #17702, .F. ) ;
#14060=VECTOR ( 'NONE', #15440, 1000.000000000000000 ) ;
#14084=CARTESIAN_POINT ( 'NONE',  ( 2.000000000000000000, 1.999999999999998224, 37.99999999999999289 ) ) ;
#14129=LINE ( 'NONE', #7824, #14060 ) ;
#14145=AXIS2_PLACEMENT_3D ( 'NONE', #10870, #1865, #11069 ) ;
#14161=ORIENTED_EDGE ( 'NONE', *, *, #2271, .T. ) ;
#14189=CARTESIAN_POINT ( 'NONE',  ( 5.000000000000000000, -2.000000000000001776, 41.99999999999999289 ) ) ;
#14198=FILL_AREA_STYLE ('',( #6674 ) ) ;
#14208=ORIENTED_EDGE ( 'NONE', *, *, #1205, .T. ) ;
#14215=CARTESIAN_POINT ( 'NONE',  ( 4.999999999999963585, 7.196152422706642682, 37.99999999999999289 ) ) ;
#14226=ORIENTED_EDGE ( 'NONE', *, *, #1214, .T. ) ;
#14251=DIRECTION ( 'NONE',  ( -0.000000000000000000, 0.000000000000000000, 1.000000000000000000 ) ) ;
#14276=FACE_OUTER_BOUND ( 'NONE', #18176, .T. ) ;
#14296=CARTESIAN_POINT ( 'NONE',  ( 8.000000000000000000, 1.999999999999997335, 37.99999999999999289 ) ) ;
#14310=ORIENTED_EDGE ( 'NONE', *, *, #13545, .F. ) ;
#14346=ORIENTED_EDGE ( 'NONE', *, *, #1010, .T. ) ;
#14373=VERTEX_POINT ( 'NONE', #19629 ) ;
#14429=CARTESIAN_POINT ( 'NONE',  ( -2.000000000000000000, -2.000000000000002665, 37.99999999999999289 ) ) ;
#14507=CARTESIAN_POINT ( 'NONE',  ( -3.207603742328077057E-13, 82.80384757729329692, 37.99999999999999289 ) ) ;
#14529=SURFACE_STYLE_FILL_AREA ( #11808 ) ;
#14542=EDGE_LOOP ( 'NONE', ( #9860, #4182, #16201, #17681 ) ) ;
#14566=CYLINDRICAL_SURFACE ( 'NONE', #3755, 3.000000000000000000 ) ;
#14576=ORIENTED_EDGE ( 'NONE', *, *, #4793, .T. ) ;
#14597=CIRCLE ( 'NONE', #13312, 3.000000000000000000 ) ;
#14625=SURFACE_STYLE_USAGE ( .BOTH. , #13114 ) ;
#14717=( LENGTH_UNIT ( ) NAMED_UNIT ( * ) SI_UNIT ( .MILLI., .METRE. ) );
#14719=CYLINDRICAL_SURFACE ( 'NONE', #15355, 6.000000000000000000 ) ;
#14726=CARTESIAN_POINT ( 'NONE',  ( -2.000000000000000000, -8.000000000000003553, 41.99999999999999289 ) ) ;
#14773=ORIENTED_EDGE ( 'NONE', *, *, #5666, .T. ) ;
#14774=VECTOR ( 'NONE', #1403, 1000.000000000000000 ) ;
#14814=LINE ( 'NONE', #10319, #4364 ) ;
#14819=ORIENTED_EDGE ( 'NONE', *, *, #18491, .T. ) ;
#14850=AXIS2_PLACEMENT_3D ( 'NONE', #10757, #8861, #5741 ) ;
#14882=ADVANCED_FACE ( 'NONE', ( #15060 ), #2943, .F. ) ;
#14884=DIRECTION ( 'NONE',  ( 0.000000000000000000, -1.000000000000000000, 0.000000000000000000 ) ) ;
#14895=DIRECTION ( 'NONE',  ( 0.000000000000000000, 0.000000000000000000, 1.000000000000000000 ) ) ;
#14974=VECTOR ( 'NONE', #19073, 1000.000000000000000 ) ;
#15013=VERTEX_POINT ( 'NONE', #18649 ) ;
#15021=VECTOR ( 'NONE', #3716, 1000.000000000000000 ) ;
#15025=DIRECTION ( 'NONE',  ( -0.000000000000000000, 0.000000000000000000, 1.000000000000000000 ) ) ;
#15030=ORIENTED_EDGE ( 'NONE', *, *, #12302, .T. ) ;
#15060=FACE_OUTER_BOUND ( 'NONE', #7247, .T. ) ;
#15064=CARTESIAN_POINT ( 'NONE',  ( -25.31088913245540084, -1.027644533213482535E-13, 41.99999999999999289 ) ) ;
#15082=CARTESIAN_POINT ( 'NONE',  ( 8.000000000000000000, 0.000000000000000000, 41.99999999999999289 ) ) ;
#15106=LINE ( 'NONE', #18209, #14774 ) ;
#15110=DIRECTION ( 'NONE',  ( 0.000000000000000000, 0.000000000000000000, 1.000000000000000000 ) ) ;
#15153=CARTESIAN_POINT ( 'NONE',  ( 8.000000000000000000, 1.999999999999997335, 37.99999999999999289 ) ) ;
#15195=ADVANCED_FACE ( 'NONE', ( #1031 ), #8453, .F. ) ;
#15239=ADVANCED_FACE ( 'NONE', ( #651 ), #940, .F. ) ;
#15276=ORIENTED_EDGE ( 'NONE', *, *, #19666, .T. ) ;
#15285=EDGE_CURVE ( 'NONE', #6248, #3602, #1530, .T. ) ;
#15318=EDGE_CURVE ( 'NONE', #9982, #9207, #18140, .T. ) ;
#15324=LINE ( 'NONE', #3107, #5355 ) ;
#15355=AXIS2_PLACEMENT_3D ( 'NONE', #14429, #6994, #5214 ) ;
#15359=ORIENTED_EDGE ( 'NONE', *, *, #4793, .F. ) ;
#15364=ORIENTED_EDGE ( 'NONE', *, *, #2441, .T. ) ;
#15385=CYLINDRICAL_SURFACE ( 'NONE', #7732, 6.000000000000000000 ) ;
#15410=ORIENTED_EDGE ( 'NONE', *, *, #4150, .F. ) ;
#15435=CARTESIAN_POINT ( 'NONE',  ( 2.000000000000000000, 1.999999999999997335, 41.99999999999999289 ) ) ;
#15440=DIRECTION ( 'NONE',  ( 0.000000000000000000, 0.000000000000000000, 1.000000000000000000 ) ) ;
#15462=ORIENTED_EDGE ( 'NONE', *, *, #8979, .T. ) ;
#15484=AXIS2_PLACEMENT_3D ( 'NONE', #3615, #3714, #11124 ) ;
#15494=EDGE_CURVE ( 'NONE', #870, #9786, #3837, .T. ) ;
#15549=VECTOR ( 'NONE', #10206, 1000.000000000000000 ) ;
#15629=ADVANCED_FACE ( 'NONE', ( #18922 ), #14719, .T. ) ;
#15643=SHAPE_REPRESENTATION ( 'brake arm', ( #16724 ), #2332 ) ;
#15666=VECTOR ( 'NONE', #6115, 1000.000000000000000 ) ;
#15670=EDGE_CURVE ( 'NONE', #6802, #10667, #8317, .T. ) ;
#15700=( LENGTH_UNIT ( ) NAMED_UNIT ( * ) SI_UNIT ( .MILLI., .METRE. ) );
#15728=DIRECTION ( 'NONE',  ( -0.000000000000000000, 0.000000000000000000, 1.000000000000000000 ) ) ;
#15759=VECTOR ( 'NONE', #13851, 1000.000000000000000 ) ;
#15767=PLANE ( 'NONE',  #16869 ) ;
#15866=CARTESIAN_POINT ( 'NONE',  ( -2.000000000000000000, -5.000000000000001776, 37.99999999999999289 ) ) ;
#15872=DIRECTION ( 'NONE',  ( -1.000000000000000000, 0.000000000000000000, 0.000000000000000000 ) ) ;
#15896=DIRECTION ( 'NONE',  ( 1.000000000000000000, 0.000000000000000000, 0.000000000000000000 ) ) ;
#15954=ORIENTED_EDGE ( 'NONE', *, *, #6737, .F. ) ;
#15990=STYLED_ITEM ( 'NONE', ( #17971 ), #16005 ) ;
#16004=DIRECTION ( 'NONE',  ( 0.000000000000000000, 0.000000000000000000, 1.000000000000000000 ) ) ;
#16005=MANIFOLD_SOLID_BREP ( 'Boss-Extrude1', #8751 ) ;
#16016=CARTESIAN_POINT ( 'NONE',  ( 8.000000000000000000, 1.999999999999997335, 41.99999999999999289 ) ) ;
#16020=( NAMED_UNIT ( * ) SI_UNIT ( $, .STERADIAN. ) SOLID_ANGLE_UNIT ( ) );
#16022=AXIS2_PLACEMENT_3D ( 'NONE', #9141, #16747, #6021 ) ;
#16023=ORIENTED_EDGE ( 'NONE', *, *, #13545, .T. ) ;
#16052=DIRECTION ( 'NONE',  ( 0.000000000000000000, 0.000000000000000000, 1.000000000000000000 ) ) ;
#16098=EDGE_CURVE ( 'NONE', #10667, #10763, #16571, .T. ) ;
#16105=( NAMED_UNIT ( * ) SI_UNIT ( $, .STERADIAN. ) SOLID_ANGLE_UNIT ( ) );
#16166=CARTESIAN_POINT ( 'NONE',  ( -39.64101615137792578, 82.80384757729314060, 37.99999999999999289 ) ) ;
#16194=LINE ( 'NONE', #8489, #817 ) ;
#16201=ORIENTED_EDGE ( 'NONE', *, *, #7528, .T. ) ;
#16212=CARTESIAN_POINT ( 'NONE',  ( 0.000000000000000000, -5.000000000000001776, 37.99999999999999289 ) ) ;
#16302=CARTESIAN_POINT ( 'NONE',  ( -39.64101615137763446, 12.80384757729311573, 37.99999999999999289 ) ) ;
#16303=CARTESIAN_POINT ( 'NONE',  ( 0.000000000000000000, 4.999999999999998224, 37.99999999999999289 ) ) ;
#16325=ORIENTED_EDGE ( 'NONE', *, *, #5657, .T. ) ;
#16396=UNCERTAINTY_MEASURE_WITH_UNIT (LENGTH_MEASURE( 1.000000000000000082E-05 ), #14717, 'distance_accuracy_value', 'NONE');
#16404=DIRECTION ( 'NONE',  ( -0.000000000000000000, 0.000000000000000000, 1.000000000000000000 ) ) ;
#16476=CARTESIAN_POINT ( 'NONE',  ( 0.000000000000000000, 4.999999999999998224, 41.99999999999999289 ) ) ;
#16483=EDGE_CURVE ( 'NONE', #18724, #5844, #14129, .T. ) ;
#16518=CARTESIAN_POINT ( 'NONE',  ( 5.000000000000000000, -2.000000000000001776, 37.99999999999999289 ) ) ;
#16571=LINE ( 'NONE', #15064, #3508 ) ;
#16580=DIRECTION ( 'NONE',  ( 4.060088635510494296E-15, -1.000000000000000000, 0.000000000000000000 ) ) ;
#16582=EDGE_LOOP ( 'NONE', ( #9665, #16325, #4853, #7499, #13675, #13752, #2942, #17811, #6528, #15359 ) ) ;
#16635=ADVANCED_FACE ( 'NONE', ( #12932, #7091 ), #19027, .T. ) ;
#16697=CIRCLE ( 'NONE', #81, 6.000000000000000000 ) ;
#16724=AXIS2_PLACEMENT_3D ( 'NONE', #17428, #9833, #6230 ) ;
#16747=DIRECTION ( 'NONE',  ( -0.000000000000000000, 0.000000000000000000, 1.000000000000000000 ) ) ;
#16756=DIRECTION ( 'NONE',  ( -0.8660254037844419273, 0.4999999999999944489, 0.000000000000000000 ) ) ;
#16781=DIRECTION ( 'NONE',  ( 1.000000000000000000, 0.000000000000000000, 0.000000000000000000 ) ) ;
#16866=VERTEX_POINT ( 'NONE', #12905 ) ;
#16869=AXIS2_PLACEMENT_3D ( 'NONE', #8355, #1948, #6734 ) ;
#16932=ADVANCED_FACE ( 'NONE', ( #11793 ), #5579, .F. ) ;
#16973=ORIENTED_EDGE ( 'NONE', *, *, #3959, .F. ) ;
#16980=LINE ( 'NONE', #648, #3641 ) ;
#16989=CARTESIAN_POINT ( 'NONE',  ( -2.000000000000000000, 4.999999999999998224, 37.99999999999999289 ) ) ;
#16999=ORIENTED_EDGE ( 'NONE', *, *, #12830, .F. ) ;
#17067=VERTEX_POINT ( 'NONE', #4681 ) ;
#17084=ORIENTED_EDGE ( 'NONE', *, *, #6063, .T. ) ;
#17136=CIRCLE ( 'NONE', #13618, 6.000000000000000000 ) ;
#17374=FACE_OUTER_BOUND ( 'NONE', #6344, .T. ) ;
#17390=AXIS2_PLACEMENT_3D ( 'NONE', #8345, #9764, #16052 ) ;
#17428=CARTESIAN_POINT ( 'NONE',  ( 0.000000000000000000, 0.000000000000000000, 0.000000000000000000 ) ) ;
#17429=PLANE ( 'NONE',  #15484 ) ;
#17525=ADVANCED_FACE ( 'NONE', ( #19600 ), #2989, .F. ) ;
#17533=PRODUCT ( 'brake arm', 'brake arm', '', ( #9661 ) ) ;
#17551=CARTESIAN_POINT ( 'NONE',  ( -2.000000000000000000, 4.999999999999998224, 41.99999999999999289 ) ) ;
#17572=ORIENTED_EDGE ( 'NONE', *, *, #16098, .T. ) ;
#17595=SURFACE_STYLE_FILL_AREA ( #14198 ) ;
#17609=FACE_OUTER_BOUND ( 'NONE', #1656, .T. ) ;
#17625=VERTEX_POINT ( 'NONE', #14189 ) ;
#17626=APPLICATION_CONTEXT ( 'automotive_design' ) ;
#17667=VECTOR ( 'NONE', #3036, 1000.000000000000000 ) ;
#17681=ORIENTED_EDGE ( 'NONE', *, *, #15285, .T. ) ;
#17686=DIRECTION ( 'NONE',  ( 0.000000000000000000, 0.000000000000000000, 1.000000000000000000 ) ) ;
#17702=EDGE_CURVE ( 'NONE', #6503, #809, #18885, .T. ) ;
#17715=CARTESIAN_POINT ( 'NONE',  ( -2.000000000000000000, -2.000000000000001776, 41.99999999999999289 ) ) ;
#17753=DIRECTION ( 'NONE',  ( 0.000000000000000000, 0.000000000000000000, 1.000000000000000000 ) ) ;
#17764=ORIENTED_EDGE ( 'NONE', *, *, #12302, .F. ) ;
#17811=ORIENTED_EDGE ( 'NONE', *, *, #16098, .F. ) ;
#17900=CARTESIAN_POINT ( 'NONE',  ( -2.000000000000000000, 1.999999999999998224, 37.99999999999999289 ) ) ;
#17911=FILL_AREA_STYLE_COLOUR ( '', #12891 ) ;
#17971=PRESENTATION_STYLE_ASSIGNMENT (( #3883 ) ) ;
#17984=LINE ( 'NONE', #10479, #10625 ) ;
#18061=CIRCLE ( 'NONE', #7502, 3.000000000000000000 ) ;
#18087=ORIENTED_EDGE ( 'NONE', *, *, #4528, .T. ) ;
#18108=CARTESIAN_POINT ( 'NONE',  ( -5.000000000000000000, 1.999999999999998668, 37.99999999999999289 ) ) ;
#18113=CARTESIAN_POINT ( 'NONE',  ( -5.000000000000000000, 0.000000000000000000, 41.99999999999999289 ) ) ;
#18138=DIRECTION ( 'NONE',  ( -1.000000000000000000, -4.060088635510494296E-15, 0.000000000000000000 ) ) ;
#18140=LINE ( 'NONE', #1229, #15666 ) ;
#18176=EDGE_LOOP ( 'NONE', ( #15954, #9268, #2434, #18087 ) ) ;
#18209=CARTESIAN_POINT ( 'NONE',  ( -5.000000000000000000, -2.000000000000001332, 37.99999999999999289 ) ) ;
#18230=ORIENTED_EDGE ( 'NONE', *, *, #399, .F. ) ;
#18317=DIRECTION ( 'NONE',  ( 0.000000000000000000, 1.000000000000000000, 0.000000000000000000 ) ) ;
#18326=VECTOR ( 'NONE', #13398, 1000.000000000000000 ) ;
#18330=ORIENTED_EDGE ( 'NONE', *, *, #5666, .F. ) ;
#18332=LINE ( 'NONE', #6012, #18977 ) ;
#18375=EDGE_CURVE ( 'NONE', #4959, #3602, #1721, .T. ) ;
#18430=DIRECTION ( 'NONE',  ( 1.000000000000000000, 0.000000000000000000, 0.000000000000000000 ) ) ;
#18460=DIRECTION ( 'NONE',  ( -0.000000000000000000, 0.000000000000000000, 1.000000000000000000 ) ) ;
#18470=FACE_OUTER_BOUND ( 'NONE', #11334, .T. ) ;
#18484=CARTESIAN_POINT ( 'NONE',  ( -2.000000000000000000, -2.000000000000002665, 37.99999999999999289 ) ) ;
#18490=DIRECTION ( 'NONE',  ( 1.000000000000000000, 0.000000000000000000, 0.000000000000000000 ) ) ;
#18491=EDGE_CURVE ( 'NONE', #11541, #12253, #18913, .T. ) ;
#18544=CARTESIAN_POINT ( 'NONE',  ( -4.999999999999966249, -7.196152422706654228, 37.99999999999999289 ) ) ;
#18548=EDGE_LOOP ( 'NONE', ( #7845, #687, #698, #16023 ) ) ;
#18551=ORIENTED_EDGE ( 'NONE', *, *, #2051, .F. ) ;
#18574=DIRECTION ( 'NONE',  ( 0.000000000000000000, 0.000000000000000000, 1.000000000000000000 ) ) ;
#18649=CARTESIAN_POINT ( 'NONE',  ( 2.000000000000000000, 4.999999999999998224, 41.99999999999999289 ) ) ;
#18655=ORIENTED_EDGE ( 'NONE', *, *, #1391, .T. ) ;
#18696=VERTEX_POINT ( 'NONE', #3807 ) ;
#18724=VERTEX_POINT ( 'NONE', #18108 ) ;
#18764=CARTESIAN_POINT ( 'NONE',  ( -25.31088913245573835, 82.80384757729319745, 37.99999999999999289 ) ) ;
#18779=EDGE_CURVE ( 'NONE', #10514, #14373, #15106, .T. ) ;
#18781=EDGE_LOOP ( 'NONE', ( #6574, #828, #18230, #15030 ) ) ;
#18799=FACE_OUTER_BOUND ( 'NONE', #161, .T. ) ;
#18806=LINE ( 'NONE', #1806, #19096 ) ;
#18836=ORIENTED_EDGE ( 'NONE', *, *, #333, .T. ) ;
#18885=CIRCLE ( 'NONE', #5465, 6.000000000000000000 ) ;
#18913=LINE ( 'NONE', #9527, #1649 ) ;
#18922=FACE_OUTER_BOUND ( 'NONE', #14542, .T. ) ;
#18977=VECTOR ( 'NONE', #9232, 1000.000000000000000 ) ;
#19000=VECTOR ( 'NONE', #16756, 1000.000000000000000 ) ;
#19027=PLANE ( 'NONE',  #5098 ) ;
#19066=AXIS2_PLACEMENT_3D ( 'NONE', #198, #4897, #10999 ) ;
#19073=DIRECTION ( 'NONE',  ( 0.000000000000000000, 0.000000000000000000, 1.000000000000000000 ) ) ;
#19096=VECTOR ( 'NONE', #11209, 1000.000000000000000 ) ;
#19158=EDGE_CURVE ( 'NONE', #870, #2904, #10485, .T. ) ;
#19168=LINE ( 'NONE', #580, #14974 ) ;
#19173=EDGE_LOOP ( 'NONE', ( #15276, #1871, #14819, #8549, #8306, #5513, #12723, #17084 ) ) ;
#19183=CARTESIAN_POINT ( 'NONE',  ( -2.000000000000000000, 4.999999999999998224, 37.99999999999999289 ) ) ;
#19207=DIRECTION ( 'NONE',  ( 1.000000000000000000, 0.000000000000000000, 0.000000000000000000 ) ) ;
#19303=CARTESIAN_POINT ( 'NONE',  ( 5.000000000000000000, 1.999999999999998224, 41.99999999999999289 ) ) ;
#19309=ORIENTED_EDGE ( 'NONE', *, *, #4528, .F. ) ;
#19313=EDGE_CURVE ( 'NONE', #12253, #17067, #6772, .T. ) ;
#19441=FACE_OUTER_BOUND ( 'NONE', #6206, .T. ) ;
#19496=LINE ( 'NONE', #7277, #18326 ) ;
#19573=ADVANCED_FACE ( 'NONE', ( #17374 ), #3659, .F. ) ;
#19600=FACE_OUTER_BOUND ( 'NONE', #2955, .T. ) ;
#19620=ORIENTED_EDGE ( 'NONE', *, *, #237, .F. ) ;
#19629=CARTESIAN_POINT ( 'NONE',  ( -5.000000000000000000, -2.000000000000001332, 41.99999999999999289 ) ) ;
#19666=EDGE_CURVE ( 'NONE', #18724, #10514, #1353, .T. ) ;
#19691=ORIENTED_EDGE ( 'NONE', *, *, #2051, .T. ) ;
#19698=CARTESIAN_POINT ( 'NONE',  ( -2.000000000000000000, -2.000000000000001776, 37.99999999999999289 ) ) ;
#19715=DIRECTION ( 'NONE',  ( -0.8660254037844419273, 0.4999999999999944489, 0.000000000000000000 ) ) ;
#19722=AXIS2_PLACEMENT_3D ( 'NONE', #7026, #17753, #13152 ) ;
#19742=ORIENTED_EDGE ( 'NONE', *, *, #4613, .T. ) ;
#19758=DIRECTION ( 'NONE',  ( 1.000000000000000000, 0.000000000000000000, 0.000000000000000000 ) ) ;
#19762=PLANE ( 'NONE',  #7838 ) ;
#19780=CARTESIAN_POINT ( 'NONE',  ( 1.999999999999998668, -8.000000000000003553, 41.99999999999999289 ) ) ;
ENDSEC;
END-ISO-10303-21;
